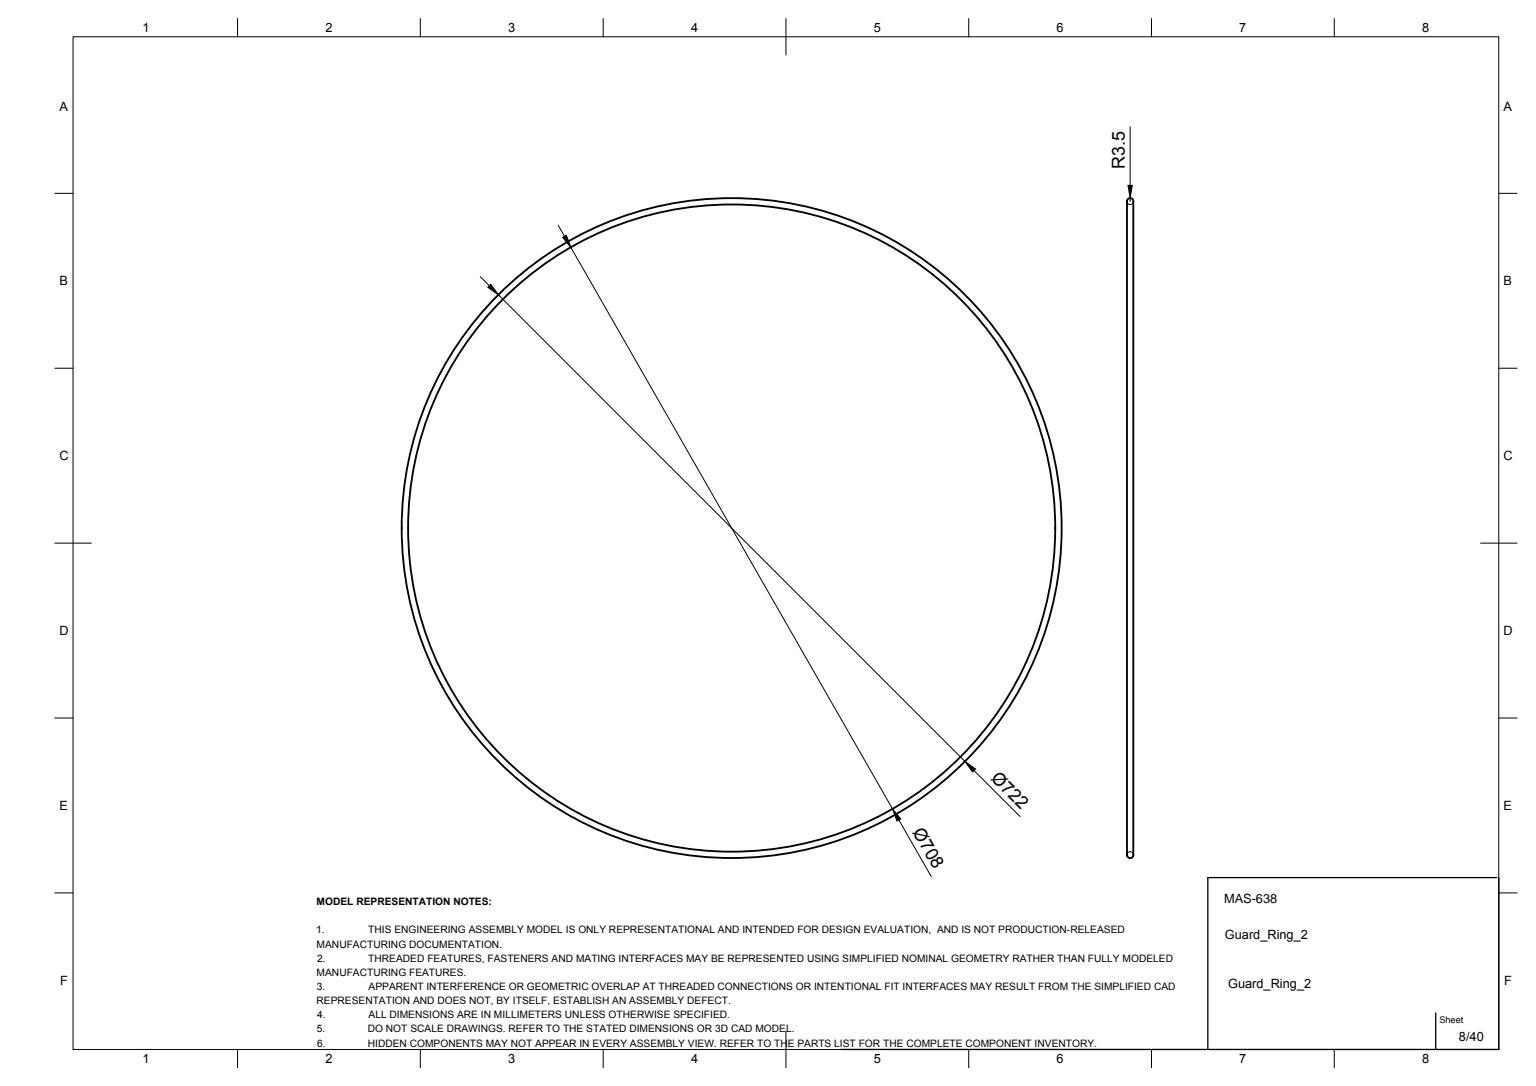
ISO-10303-21;
HEADER;
FILE_DESCRIPTION((''),'2;1');
FILE_NAME('Guard_Ring_2.step','2026-10-09T12:00:21-07:00',(''),(''),'','','');
FILE_SCHEMA (('AUTOMOTIVE_DESIGN { 1 0 10303 214 3 1 1 }'));
ENDSEC;
DATA;
#10=MECHANICAL_DESIGN_GEOMETRIC_PRESENTATION_REPRESENTATION('',(#399),#10334);
#335=SHAPE_REPRESENTATION_RELATIONSHIP('SRR','None',#10451,#367) ;
#367=ADVANCED_BREP_SHAPE_REPRESENTATION('',(#439),#10303) ;
#399=STYLED_ITEM('',(#10631),#439) ;
#439=MANIFOLD_SOLID_BREP('Body1',#3561) ;
#860=FACE_OUTER_BOUND('',#1060,.T.) ;
#1060=EDGE_LOOP('',(#2353,#2354,#2355,#2356)) ;
#1278=CIRCLE('',#3979,0.349999999999999) ;
#1279=CIRCLE('',#3980,35.4) ;
#1514=VERTEX_POINT('',#5658) ;
#1833=EDGE_CURVE('',#1514,#1514,#1278,.T.) ;
#1834=EDGE_CURVE('',#1514,#1514,#1279,.T.) ;
#2353=ORIENTED_EDGE('',*,*,#1833,.F.) ;
#2354=ORIENTED_EDGE('',*,*,#1834,.T.) ;
#2355=ORIENTED_EDGE('',*,*,#1833,.T.) ;
#2356=ORIENTED_EDGE('',*,*,#1834,.F.) ;
#3306=TOROIDAL_SURFACE('',#3978,35.75,0.349999999999999) ;
#3368=ADVANCED_FACE('',(#860),#3306,.T.) ;
#3561=CLOSED_SHELL('',(#3368)) ;
#3977=AXIS2_PLACEMENT_3D('',#5656,#4515,#4516) ;
#3978=AXIS2_PLACEMENT_3D('',#5657,#4517,#4518) ;
#3979=AXIS2_PLACEMENT_3D('',#5659,#4519,#4520) ;
#3980=AXIS2_PLACEMENT_3D('',#5660,#4521,#4522) ;
#4515=DIRECTION('axis',(0.,0.,1.)) ;
#4516=DIRECTION('refdir',(1.,0.,0.)) ;
#4517=DIRECTION('center_axis',(6.42891162084177E-17,1.,1.01883556321148E-16)) ;
#4518=DIRECTION('ref_axis',(-1.,0.,0.)) ;
#4519=DIRECTION('center_axis',(0.,1.01883556321148E-16,-1.)) ;
#4520=DIRECTION('ref_axis',(1.,0.,0.)) ;
#4521=DIRECTION('center_axis',(-6.42891162084177E-17,-1.,-1.01883556321148E-16)) ;
#4522=DIRECTION('ref_axis',(-1.,6.42891162084177E-17,6.55000379205715E-33)) ;
#5656=CARTESIAN_POINT('',(0.,0.,0.)) ;
#5657=CARTESIAN_POINT('Origin',(23.47768801576,61.7830586252741,68.2224337400009)) ;
#5658=CARTESIAN_POINT('',(58.87768801576,61.7830586252741,68.2224337400009)) ;
#5659=CARTESIAN_POINT('Origin',(59.22768801576,61.7830586252741,68.2224337400009)) ;
#5660=CARTESIAN_POINT('Origin',(23.47768801576,61.7830586252741,68.2224337400009)) ;
#10266=UNCERTAINTY_MEASURE_WITH_UNIT(LENGTH_MEASURE(0.001),#10335,
'DISTANCE_ACCURACY_VALUE',
'Maximum model space distance between geometric entities at asserted c
onnectivities') ;
#10297=UNCERTAINTY_MEASURE_WITH_UNIT(LENGTH_MEASURE(0.001),#10335,
'DISTANCE_ACCURACY_VALUE',
'Maximum model space distance between geometric entities at asserted c
onnectivities') ;
#10303=(
GEOMETRIC_REPRESENTATION_CONTEXT(3)
GLOBAL_UNCERTAINTY_ASSIGNED_CONTEXT((#10266))
GLOBAL_UNIT_ASSIGNED_CONTEXT((#10335,#10337,#10338))
REPRESENTATION_CONTEXT('','3D')
) ;
#10334=(
GEOMETRIC_REPRESENTATION_CONTEXT(3)
GLOBAL_UNCERTAINTY_ASSIGNED_CONTEXT((#10297))
GLOBAL_UNIT_ASSIGNED_CONTEXT((#10335,#10337,#10338))
REPRESENTATION_CONTEXT('','3D')
) ;
#10335=(
LENGTH_UNIT()
NAMED_UNIT(*)
SI_UNIT(.CENTI.,.METRE.)
) ;
#10337=(
NAMED_UNIT(*)
PLANE_ANGLE_UNIT()
SI_UNIT($,.RADIAN.)
) ;
#10338=(
NAMED_UNIT(*)
SI_UNIT($,.STERADIAN.)
SOLID_ANGLE_UNIT()
) ;
#10344=SHAPE_DEFINITION_REPRESENTATION(#10380,#10451) ;
#10380=PRODUCT_DEFINITION_SHAPE('',$,#10488) ;
#10451=SHAPE_REPRESENTATION('',(#3977),#10303) ;
#10482=PRODUCT_DEFINITION_CONTEXT('part definition',#10592,'design') ;
#10488=PRODUCT_DEFINITION('Guard_Ring_2','Guard_Ring_2',#10524,#10482) ;
#10524=PRODUCT_DEFINITION_FORMATION('',$,#10599) ;
#10592=APPLICATION_CONTEXT(
'Core Data for Automotive Mechanical Design Process') ;
#10593=PRODUCT_CONTEXT('part definition',#10592,'mechanical') ;
#10599=PRODUCT('Guard_Ring_2','Guard_Ring_2',$,(#10593)) ;
#10631=PRESENTATION_STYLE_ASSIGNMENT((#10635)) ;
#10635=SURFACE_STYLE_USAGE(.BOTH.,#10639) ;
#10639=SURFACE_SIDE_STYLE('',(#10643)) ;
#10643=SURFACE_STYLE_FILL_AREA(#10647) ;
#10647=FILL_AREA_STYLE('Opaque(25,25,25)',(#10651)) ;
#10651=FILL_AREA_STYLE_COLOUR('Opaque(25,25,25)',#10655) ;
#10655=COLOUR_RGB('Opaque(25,25,25)', 0.09019608, 0.27058824, 0.51372549) ;
ENDSEC;
END-ISO-10303-21;
